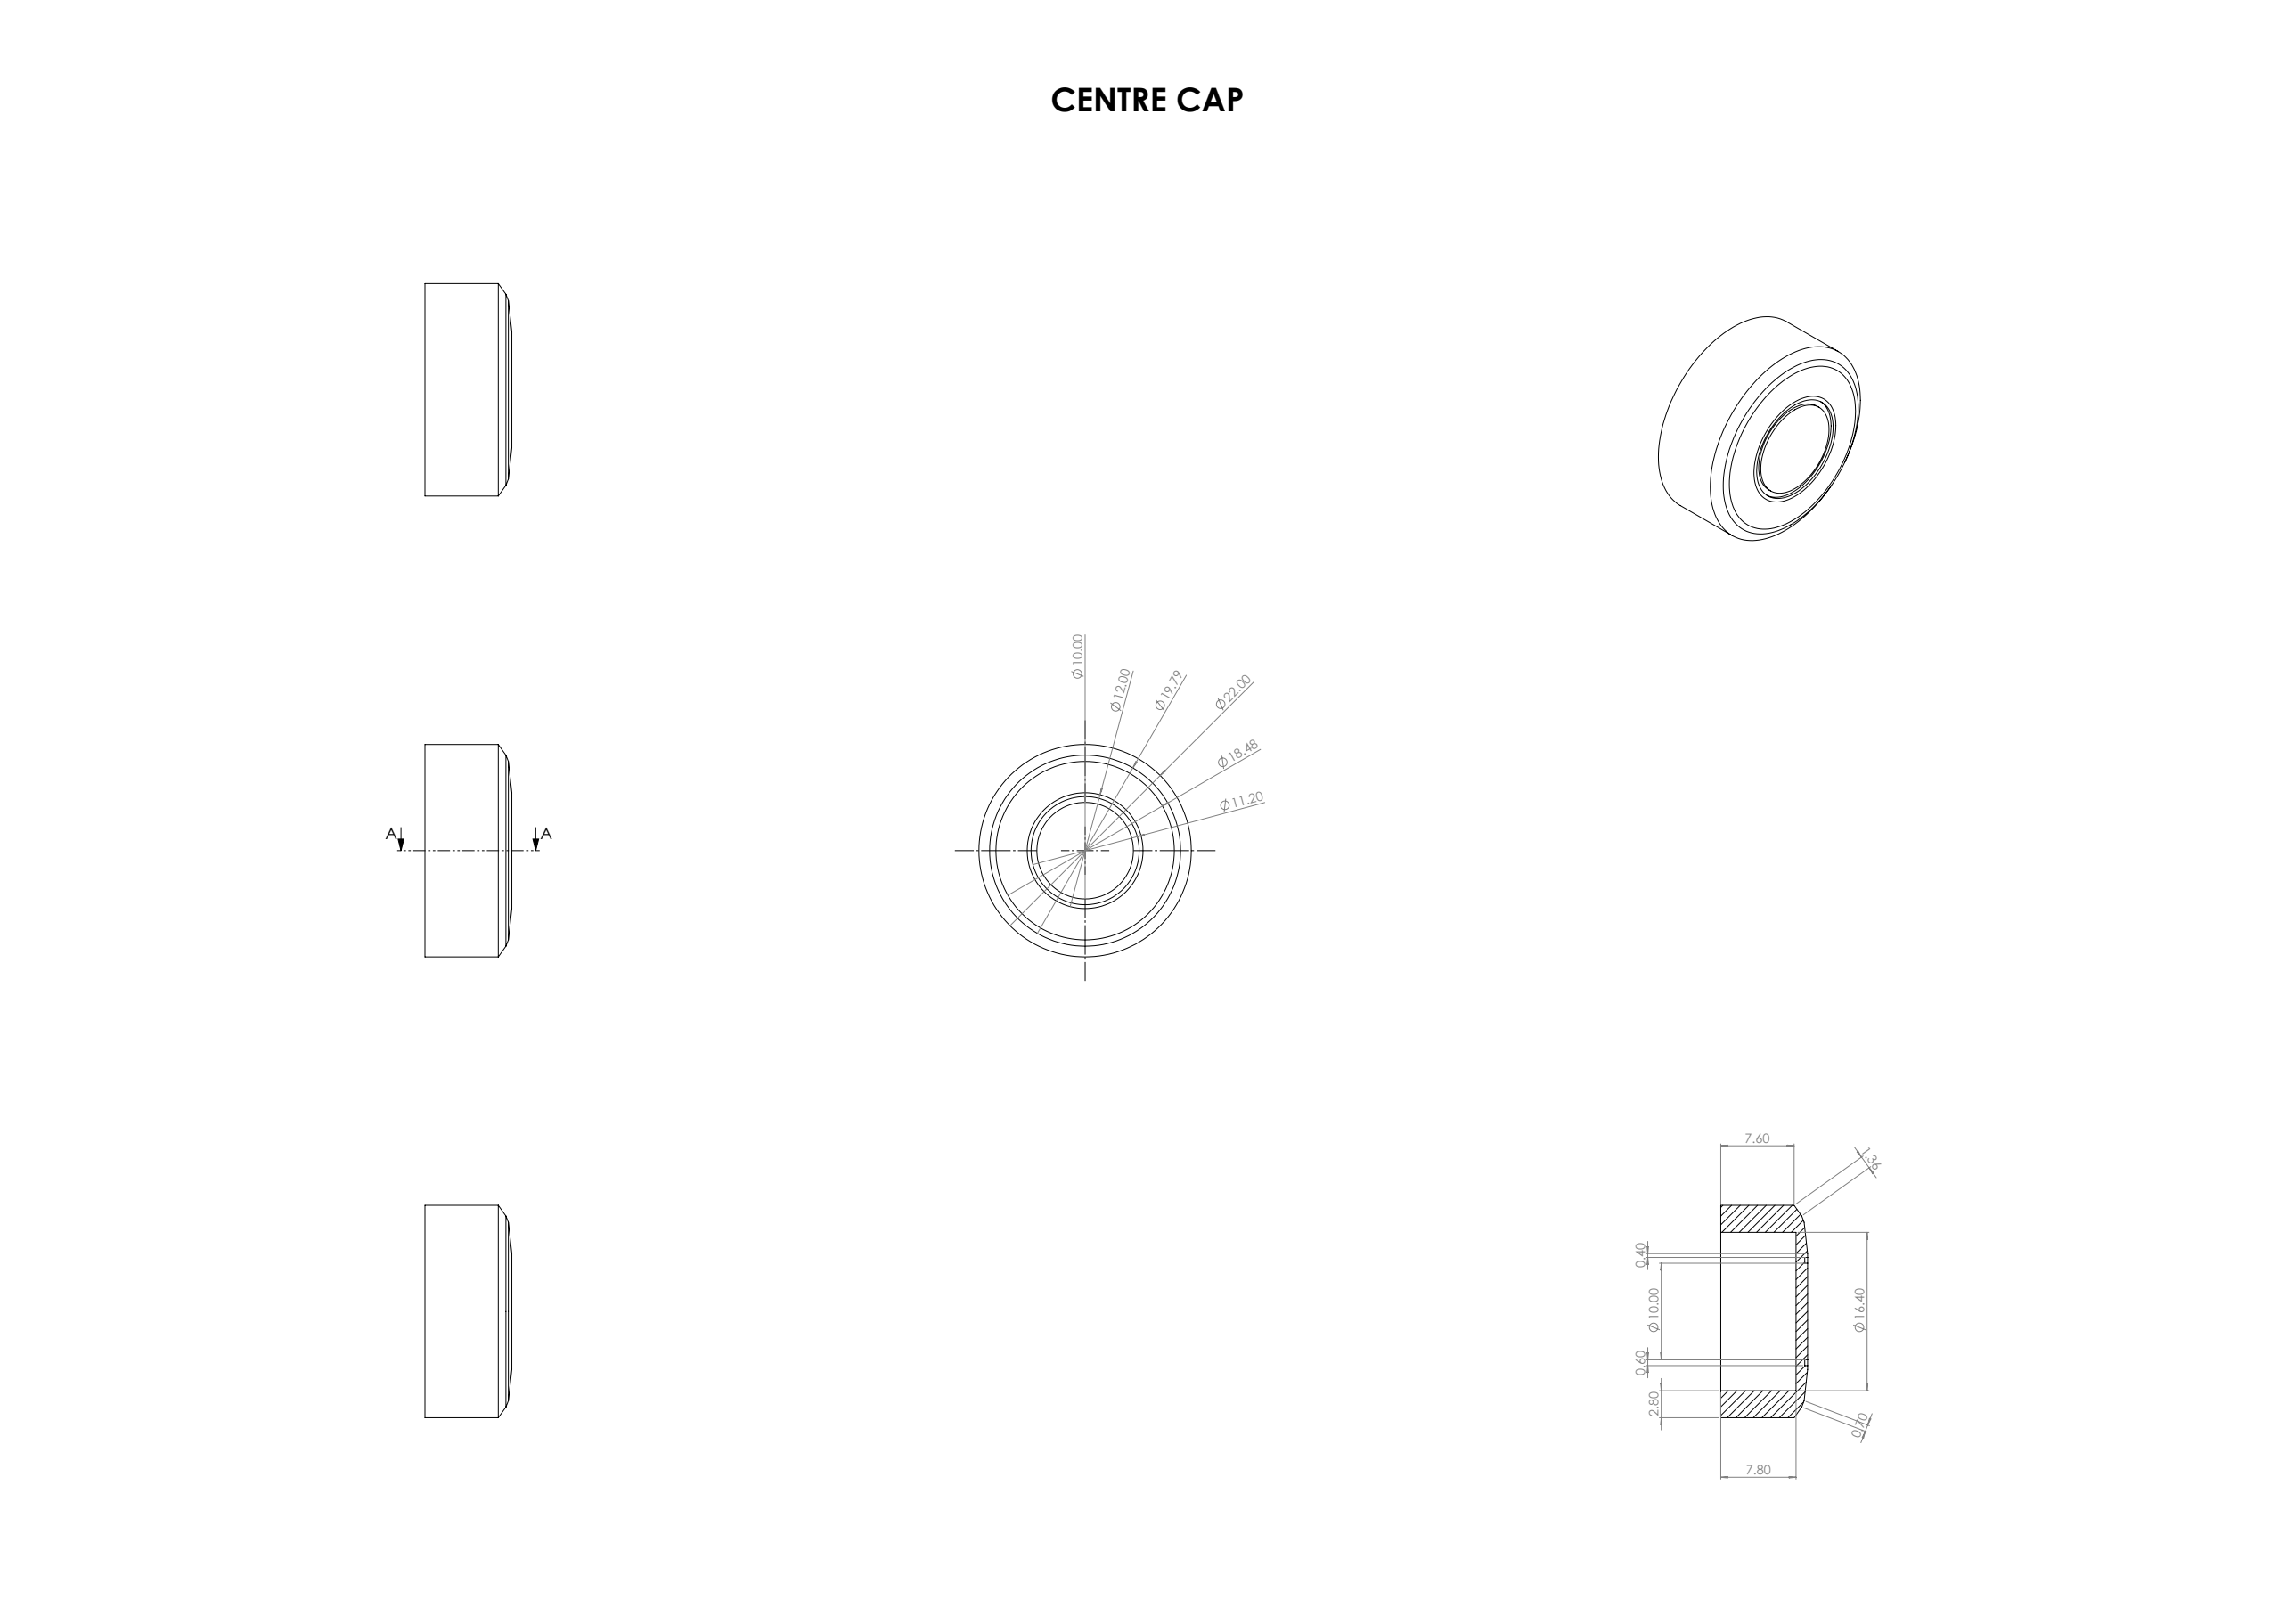
ISO-10303-21;
HEADER;
/* Generated by software containing ST-Developer
 * from STEP Tools, Inc. (www.steptools.com) 
 */

FILE_DESCRIPTION(
/* description */ (''),
/* implementation_level */ '2;1');

FILE_NAME(
/* name */ '05_Centre_Cap.step',
/* time_stamp */ '2026-10-21T02:03:06-07:00',
/* author */ (''),
/* organization */ (''),
/* preprocessor_version */ 'ST-DEVELOPER v20.2',
/* originating_system */ 'Autodesk Translation Framework v15.15.0.0',
/* authorisation */ '');

FILE_SCHEMA (('AUTOMOTIVE_DESIGN { 1 0 10303 214 3 1 1 }'));
ENDSEC;

DATA;
#10=MECHANICAL_DESIGN_GEOMETRIC_PRESENTATION_REPRESENTATION('',(#119),#38528);
#95=SHAPE_REPRESENTATION_RELATIONSHIP('SRR','None',#38580,#107);
#107=ADVANCED_BREP_SHAPE_REPRESENTATION('',(#131),#38520);
#119=STYLED_ITEM('',(#38692),#131);
#131=MANIFOLD_SOLID_BREP('Body1',#17076);
#377=CYLINDRICAL_SURFACE('',#18686,5.6);
#378=CYLINDRICAL_SURFACE('',#18688,5.);
#379=CYLINDRICAL_SURFACE('',#18691,8.2);
#380=CYLINDRICAL_SURFACE('',#18696,11.);
#1031=CONICAL_SURFACE('',#18674,9.56757295257596,1.20534297321654);
#1032=CONICAL_SURFACE('',#18679,10.3,0.950546840812076);
#1033=CONICAL_SURFACE('',#18681,7.8,1.460139105621);
#1466=FACE_BOUND('',#4065,.T.);
#1467=FACE_BOUND('',#4071,.T.);
#1468=FACE_BOUND('',#4074,.T.);
#2160=CIRCLE('',#18675,9.2422018555175);
#2161=CIRCLE('',#18676,9.2422018555175);
#2162=CIRCLE('',#18677,9.89294404963443);
#2163=CIRCLE('',#18678,9.89294404963443);
#2164=CIRCLE('',#18680,11.);
#2165=CIRCLE('',#18682,6.);
#2166=CIRCLE('',#18684,5.6);
#2167=CIRCLE('',#18685,5.);
#2168=CIRCLE('',#18687,5.6);
#2169=CIRCLE('',#18689,5.);
#2170=CIRCLE('',#18692,8.2);
#2171=CIRCLE('',#18693,8.2);
#2172=CIRCLE('',#18695,11.);
#3044=FACE_OUTER_BOUND('',#4061,.T.);
#3045=FACE_OUTER_BOUND('',#4062,.T.);
#3046=FACE_OUTER_BOUND('',#4063,.T.);
#3047=FACE_OUTER_BOUND('',#4064,.T.);
#3048=FACE_OUTER_BOUND('',#4066,.T.);
#3049=FACE_OUTER_BOUND('',#4067,.T.);
#3050=FACE_OUTER_BOUND('',#4068,.T.);
#3051=FACE_OUTER_BOUND('',#4069,.T.);
#3052=FACE_OUTER_BOUND('',#4070,.T.);
#3053=FACE_OUTER_BOUND('',#4072,.T.);
#3054=FACE_OUTER_BOUND('',#4073,.T.);
#3055=FACE_OUTER_BOUND('',#4075,.T.);
#4061=EDGE_LOOP('',(#14479,#14480,#14481,#14482,#14483,#14484));
#4062=EDGE_LOOP('',(#14485,#14486,#14487,#14488,#14489));
#4063=EDGE_LOOP('',(#14490,#14491,#14492,#14493,#14494));
#4064=EDGE_LOOP('',(#14495));
#4065=EDGE_LOOP('',(#14496));
#4066=EDGE_LOOP('',(#14497,#14498,#14499,#14500));
#4067=EDGE_LOOP('',(#14501,#14502,#14503,#14504));
#4068=EDGE_LOOP('',(#14505));
#4069=EDGE_LOOP('',(#14506,#14507,#14508,#14509));
#4070=EDGE_LOOP('',(#14510));
#4071=EDGE_LOOP('',(#14511));
#4072=EDGE_LOOP('',(#14512,#14513,#14514,#14515));
#4073=EDGE_LOOP('',(#14516));
#4074=EDGE_LOOP('',(#14517));
#4075=EDGE_LOOP('',(#14518));
#5019=LINE('',#33126,#5994);
#5020=LINE('',#33132,#5995);
#5021=LINE('',#33137,#5996);
#5022=LINE('',#33145,#5997);
#5023=LINE('',#33149,#5998);
#5024=LINE('',#33156,#5999);
#5025=LINE('',#33162,#6000);
#5994=VECTOR('',#22673,9.56757295257596);
#5995=VECTOR('',#22680,10.3);
#5996=VECTOR('',#22687,7.8);
#5997=VECTOR('',#22696,5.6);
#5998=VECTOR('',#22701,5.);
#5999=VECTOR('',#22710,8.2);
#6000=VECTOR('',#22719,11.);
#7511=VERTEX_POINT('',#33121);
#7512=VERTEX_POINT('',#33122);
#7513=VERTEX_POINT('',#33125);
#7514=VERTEX_POINT('',#33127);
#7515=VERTEX_POINT('',#33131);
#7516=VERTEX_POINT('',#33135);
#7517=VERTEX_POINT('',#33139);
#7518=VERTEX_POINT('',#33141);
#7519=VERTEX_POINT('',#33144);
#7520=VERTEX_POINT('',#33148);
#7521=VERTEX_POINT('',#33153);
#7522=VERTEX_POINT('',#33155);
#7523=VERTEX_POINT('',#33159);
#9891=EDGE_CURVE('',#7511,#7512,#2160,.T.);
#9892=EDGE_CURVE('',#7512,#7511,#2161,.T.);
#9893=EDGE_CURVE('',#7511,#7513,#5019,.T.);
#9894=EDGE_CURVE('',#7513,#7514,#2162,.T.);
#9895=EDGE_CURVE('',#7514,#7513,#2163,.T.);
#9896=EDGE_CURVE('',#7514,#7515,#5020,.T.);
#9897=EDGE_CURVE('',#7515,#7515,#2164,.T.);
#9898=EDGE_CURVE('',#7516,#7516,#2165,.T.);
#9899=EDGE_CURVE('',#7516,#7512,#5021,.T.);
#9900=EDGE_CURVE('',#7517,#7517,#2166,.T.);
#9901=EDGE_CURVE('',#7518,#7518,#2167,.T.);
#9902=EDGE_CURVE('',#7517,#7519,#5022,.T.);
#9903=EDGE_CURVE('',#7519,#7519,#2168,.T.);
#9904=EDGE_CURVE('',#7518,#7520,#5023,.T.);
#9905=EDGE_CURVE('',#7520,#7520,#2169,.T.);
#9906=EDGE_CURVE('',#7521,#7521,#2170,.T.);
#9907=EDGE_CURVE('',#7521,#7522,#5024,.T.);
#9908=EDGE_CURVE('',#7522,#7522,#2171,.T.);
#9909=EDGE_CURVE('',#7523,#7523,#2172,.T.);
#9910=EDGE_CURVE('',#7515,#7523,#5025,.T.);
#14479=ORIENTED_EDGE('',*,*,#9891,.T.);
#14480=ORIENTED_EDGE('',*,*,#9892,.T.);
#14481=ORIENTED_EDGE('',*,*,#9893,.T.);
#14482=ORIENTED_EDGE('',*,*,#9894,.T.);
#14483=ORIENTED_EDGE('',*,*,#9895,.T.);
#14484=ORIENTED_EDGE('',*,*,#9893,.F.);
#14485=ORIENTED_EDGE('',*,*,#9894,.F.);
#14486=ORIENTED_EDGE('',*,*,#9895,.F.);
#14487=ORIENTED_EDGE('',*,*,#9896,.T.);
#14488=ORIENTED_EDGE('',*,*,#9897,.T.);
#14489=ORIENTED_EDGE('',*,*,#9896,.F.);
#14490=ORIENTED_EDGE('',*,*,#9898,.F.);
#14491=ORIENTED_EDGE('',*,*,#9899,.T.);
#14492=ORIENTED_EDGE('',*,*,#9891,.F.);
#14493=ORIENTED_EDGE('',*,*,#9892,.F.);
#14494=ORIENTED_EDGE('',*,*,#9899,.F.);
#14495=ORIENTED_EDGE('',*,*,#9900,.T.);
#14496=ORIENTED_EDGE('',*,*,#9901,.F.);
#14497=ORIENTED_EDGE('',*,*,#9900,.F.);
#14498=ORIENTED_EDGE('',*,*,#9902,.T.);
#14499=ORIENTED_EDGE('',*,*,#9903,.F.);
#14500=ORIENTED_EDGE('',*,*,#9902,.F.);
#14501=ORIENTED_EDGE('',*,*,#9901,.T.);
#14502=ORIENTED_EDGE('',*,*,#9904,.T.);
#14503=ORIENTED_EDGE('',*,*,#9905,.F.);
#14504=ORIENTED_EDGE('',*,*,#9904,.F.);
#14505=ORIENTED_EDGE('',*,*,#9905,.T.);
#14506=ORIENTED_EDGE('',*,*,#9906,.T.);
#14507=ORIENTED_EDGE('',*,*,#9907,.T.);
#14508=ORIENTED_EDGE('',*,*,#9908,.F.);
#14509=ORIENTED_EDGE('',*,*,#9907,.F.);
#14510=ORIENTED_EDGE('',*,*,#9909,.F.);
#14511=ORIENTED_EDGE('',*,*,#9908,.T.);
#14512=ORIENTED_EDGE('',*,*,#9897,.F.);
#14513=ORIENTED_EDGE('',*,*,#9910,.T.);
#14514=ORIENTED_EDGE('',*,*,#9909,.T.);
#14515=ORIENTED_EDGE('',*,*,#9910,.F.);
#14516=ORIENTED_EDGE('',*,*,#9898,.T.);
#14517=ORIENTED_EDGE('',*,*,#9903,.T.);
#14518=ORIENTED_EDGE('',*,*,#9906,.F.);
#15953=PLANE('',#18683);
#15954=PLANE('',#18690);
#15955=PLANE('',#18694);
#15956=PLANE('',#18697);
#15957=PLANE('',#18698);
#16853=ADVANCED_FACE('',(#3044),#1031,.T.);
#16854=ADVANCED_FACE('',(#3045),#1032,.T.);
#16855=ADVANCED_FACE('',(#3046),#1033,.T.);
#16856=ADVANCED_FACE('',(#3047,#1466),#15953,.F.);
#16857=ADVANCED_FACE('',(#3048),#377,.F.);
#16858=ADVANCED_FACE('',(#3049),#378,.T.);
#16859=ADVANCED_FACE('',(#3050),#15954,.T.);
#16860=ADVANCED_FACE('',(#3051),#379,.F.);
#16861=ADVANCED_FACE('',(#3052,#1467),#15955,.T.);
#16862=ADVANCED_FACE('',(#3053),#380,.T.);
#16863=ADVANCED_FACE('',(#3054,#1468),#15956,.T.);
#16864=ADVANCED_FACE('',(#3055),#15957,.T.);
#17076=CLOSED_SHELL('',(#16853,#16854,#16855,#16856,#16857,#16858,#16859,
#16860,#16861,#16862,#16863,#16864));
#18673=AXIS2_PLACEMENT_3D('',#33119,#22665,#22666);
#18674=AXIS2_PLACEMENT_3D('',#33120,#22667,#22668);
#18675=AXIS2_PLACEMENT_3D('',#33123,#22669,#22670);
#18676=AXIS2_PLACEMENT_3D('',#33124,#22671,#22672);
#18677=AXIS2_PLACEMENT_3D('',#33128,#22674,#22675);
#18678=AXIS2_PLACEMENT_3D('',#33129,#22676,#22677);
#18679=AXIS2_PLACEMENT_3D('',#33130,#22678,#22679);
#18680=AXIS2_PLACEMENT_3D('',#33133,#22681,#22682);
#18681=AXIS2_PLACEMENT_3D('',#33134,#22683,#22684);
#18682=AXIS2_PLACEMENT_3D('',#33136,#22685,#22686);
#18683=AXIS2_PLACEMENT_3D('',#33138,#22688,#22689);
#18684=AXIS2_PLACEMENT_3D('',#33140,#22690,#22691);
#18685=AXIS2_PLACEMENT_3D('',#33142,#22692,#22693);
#18686=AXIS2_PLACEMENT_3D('',#33143,#22694,#22695);
#18687=AXIS2_PLACEMENT_3D('',#33146,#22697,#22698);
#18688=AXIS2_PLACEMENT_3D('',#33147,#22699,#22700);
#18689=AXIS2_PLACEMENT_3D('',#33150,#22702,#22703);
#18690=AXIS2_PLACEMENT_3D('',#33151,#22704,#22705);
#18691=AXIS2_PLACEMENT_3D('',#33152,#22706,#22707);
#18692=AXIS2_PLACEMENT_3D('',#33154,#22708,#22709);
#18693=AXIS2_PLACEMENT_3D('',#33157,#22711,#22712);
#18694=AXIS2_PLACEMENT_3D('',#33158,#22713,#22714);
#18695=AXIS2_PLACEMENT_3D('',#33160,#22715,#22716);
#18696=AXIS2_PLACEMENT_3D('',#33161,#22717,#22718);
#18697=AXIS2_PLACEMENT_3D('',#33163,#22720,#22721);
#18698=AXIS2_PLACEMENT_3D('',#33164,#22722,#22723);
#22665=DIRECTION('axis',(0.,0.,1.));
#22666=DIRECTION('refdir',(1.,0.,0.));
#22667=DIRECTION('center_axis',(-1.,0.,-1.6002526653361E-16));
#22668=DIRECTION('ref_axis',(0.,-1.,-6.12323399573677E-17));
#22669=DIRECTION('center_axis',(-1.,0.,0.));
#22670=DIRECTION('ref_axis',(0.,-1.,-6.12323399573677E-17));
#22671=DIRECTION('center_axis',(-1.,0.,0.));
#22672=DIRECTION('ref_axis',(0.,-1.,-6.12323399573677E-17));
#22673=DIRECTION('',(-0.35737274613036,0.933961840935295,1.14377337902718E-16));
#22674=DIRECTION('center_axis',(1.,0.,0.));
#22675=DIRECTION('ref_axis',(0.,-1.,-6.12323399573676E-17));
#22676=DIRECTION('center_axis',(1.,0.,0.));
#22677=DIRECTION('ref_axis',(0.,-1.,-6.12323399573676E-17));
#22678=DIRECTION('center_axis',(-1.,0.,0.));
#22679=DIRECTION('ref_axis',(0.,1.,0.));
#22680=DIRECTION('',(-0.581238193719096,-0.813733471206735,-9.96536090872393E-17));
#22681=DIRECTION('center_axis',(1.,0.,0.));
#22682=DIRECTION('ref_axis',(0.,0.,-1.));
#22683=DIRECTION('center_axis',(-1.,0.,0.));
#22684=DIRECTION('ref_axis',(0.,1.,0.));
#22685=DIRECTION('center_axis',(1.,0.,0.));
#22686=DIRECTION('ref_axis',(0.,0.,-1.));
#22687=DIRECTION('',(-0.110431526074847,-0.993883734673619,-1.21715653439266E-16));
#22688=DIRECTION('center_axis',(-1.,0.,0.));
#22689=DIRECTION('ref_axis',(0.,0.,1.));
#22690=DIRECTION('center_axis',(1.,0.,0.));
#22691=DIRECTION('ref_axis',(0.,0.,-1.));
#22692=DIRECTION('center_axis',(1.,0.,0.));
#22693=DIRECTION('ref_axis',(0.,0.,-1.));
#22694=DIRECTION('center_axis',(1.,0.,0.));
#22695=DIRECTION('ref_axis',(0.,1.,0.));
#22696=DIRECTION('',(1.,0.,0.));
#22697=DIRECTION('center_axis',(-1.,0.,0.));
#22698=DIRECTION('ref_axis',(0.,1.,0.));
#22699=DIRECTION('center_axis',(1.,0.,0.));
#22700=DIRECTION('ref_axis',(0.,1.,0.));
#22701=DIRECTION('',(1.,0.,0.));
#22702=DIRECTION('center_axis',(1.,0.,0.));
#22703=DIRECTION('ref_axis',(0.,1.,0.));
#22704=DIRECTION('center_axis',(1.,0.,0.));
#22705=DIRECTION('ref_axis',(0.,0.,-1.));
#22706=DIRECTION('center_axis',(1.,0.,0.));
#22707=DIRECTION('ref_axis',(0.,1.,0.));
#22708=DIRECTION('center_axis',(1.,0.,0.));
#22709=DIRECTION('ref_axis',(0.,0.,-1.));
#22710=DIRECTION('',(-1.,0.,0.));
#22711=DIRECTION('center_axis',(1.,0.,0.));
#22712=DIRECTION('ref_axis',(0.,0.,-1.));
#22713=DIRECTION('center_axis',(-1.,0.,0.));
#22714=DIRECTION('ref_axis',(0.,0.,1.));
#22715=DIRECTION('center_axis',(1.,0.,0.));
#22716=DIRECTION('ref_axis',(0.,0.,-1.));
#22717=DIRECTION('center_axis',(1.,0.,0.));
#22718=DIRECTION('ref_axis',(0.,1.,0.));
#22719=DIRECTION('',(-1.,0.,0.));
#22720=DIRECTION('center_axis',(1.,0.,0.));
#22721=DIRECTION('ref_axis',(0.,0.,-1.));
#22722=DIRECTION('center_axis',(-1.,0.,0.));
#22723=DIRECTION('ref_axis',(0.,0.,1.));
#33119=CARTESIAN_POINT('',(0.,0.,0.));
#33120=CARTESIAN_POINT('Origin',(8.51525479982404,0.,-5.85844879599047E-16));
#33121=CARTESIAN_POINT('',(8.63975534938695,9.2422018555175,-1.13184329194332E-15));
#33122=CARTESIAN_POINT('',(8.63975534938694,-9.2422018555175,-1.13184329194332E-15));
#33123=CARTESIAN_POINT('Origin',(8.63975534938695,0.,-5.65921645971662E-16));
#33124=CARTESIAN_POINT('Origin',(8.63975534938695,0.,-5.65921645971662E-16));
#33125=CARTESIAN_POINT('',(8.39075425026112,9.89294404963443,1.21153622645287E-15));
#33126=CARTESIAN_POINT('',(8.51525479982404,9.56757295257596,1.17168975919809E-15));
#33127=CARTESIAN_POINT('',(8.39075425026113,-9.89294404963442,-1.21153622645287E-15));
#33128=CARTESIAN_POINT('Origin',(8.39075425026112,0.,-6.05768113226433E-16));
#33129=CARTESIAN_POINT('Origin',(8.39075425026112,0.,-6.05768113226433E-16));
#33130=CARTESIAN_POINT('Origin',(8.1,0.,0.));
#33131=CARTESIAN_POINT('',(7.6,-11.,-1.34711147906209E-15));
#33132=CARTESIAN_POINT('',(8.1,-10.3,-1.26138620312177E-15));
#33133=CARTESIAN_POINT('Origin',(7.6,0.,0.));
#33134=CARTESIAN_POINT('Origin',(8.8,0.,0.));
#33135=CARTESIAN_POINT('',(9.,-6.,-7.34788079488412E-16));
#33136=CARTESIAN_POINT('Origin',(9.,0.,0.));
#33137=CARTESIAN_POINT('',(8.8,-7.8,-9.55224503334935E-16));
#33138=CARTESIAN_POINT('Origin',(8.7,5.6,0.));
#33139=CARTESIAN_POINT('',(8.7,-5.6,-6.85802207522518E-16));
#33140=CARTESIAN_POINT('Origin',(8.7,0.,0.));
#33141=CARTESIAN_POINT('',(8.7,-5.,-6.12323399573677E-16));
#33142=CARTESIAN_POINT('Origin',(8.7,0.,0.));
#33143=CARTESIAN_POINT('Origin',(8.855,0.,0.));
#33144=CARTESIAN_POINT('',(9.,-5.6,6.85802207522518E-16));
#33145=CARTESIAN_POINT('',(8.855,-5.6,-6.85802207522518E-16));
#33146=CARTESIAN_POINT('Origin',(9.,0.,0.));
#33147=CARTESIAN_POINT('Origin',(8.855,0.,0.));
#33148=CARTESIAN_POINT('',(9.,-5.,-6.12323399573677E-16));
#33149=CARTESIAN_POINT('',(8.855,-5.,-6.12323399573677E-16));
#33150=CARTESIAN_POINT('Origin',(9.,0.,0.));
#33151=CARTESIAN_POINT('Origin',(9.,0.,0.));
#33152=CARTESIAN_POINT('Origin',(3.9,0.,0.));
#33153=CARTESIAN_POINT('',(7.8,-8.2,-1.00421037530083E-15));
#33154=CARTESIAN_POINT('Origin',(7.8,0.,0.));
#33155=CARTESIAN_POINT('',(0.,-8.2,-1.00421037530083E-15));
#33156=CARTESIAN_POINT('',(3.9,-8.2,-1.00421037530083E-15));
#33157=CARTESIAN_POINT('Origin',(0.,0.,0.));
#33158=CARTESIAN_POINT('Origin',(0.,11.,0.));
#33159=CARTESIAN_POINT('',(5.55111512312578E-16,-11.,-1.34711147906209E-15));
#33160=CARTESIAN_POINT('Origin',(0.,0.,0.));
#33161=CARTESIAN_POINT('Origin',(3.8,0.,0.));
#33162=CARTESIAN_POINT('',(3.8,-11.,-1.34711147906209E-15));
#33163=CARTESIAN_POINT('Origin',(9.,0.,0.));
#33164=CARTESIAN_POINT('Origin',(7.8,8.2,0.));
#38506=UNCERTAINTY_MEASURE_WITH_UNIT(LENGTH_MEASURE(0.01),#38529,
'DISTANCE_ACCURACY_VALUE',
'Maximum model space distance between geometric entities at asserted c
onnectivities');
#38514=UNCERTAINTY_MEASURE_WITH_UNIT(LENGTH_MEASURE(0.01),#38529,
'DISTANCE_ACCURACY_VALUE',
'Maximum model space distance between geometric entities at asserted c
onnectivities');
#38520=(
GEOMETRIC_REPRESENTATION_CONTEXT(3)
GLOBAL_UNCERTAINTY_ASSIGNED_CONTEXT((#38506))
GLOBAL_UNIT_ASSIGNED_CONTEXT((#38529,#38531,#38532))
REPRESENTATION_CONTEXT('','3D')
);
#38528=(
GEOMETRIC_REPRESENTATION_CONTEXT(3)
GLOBAL_UNCERTAINTY_ASSIGNED_CONTEXT((#38514))
GLOBAL_UNIT_ASSIGNED_CONTEXT((#38529,#38531,#38532))
REPRESENTATION_CONTEXT('','3D')
);
#38529=(
LENGTH_UNIT()
NAMED_UNIT(*)
SI_UNIT(.MILLI.,.METRE.)
);
#38531=(
NAMED_UNIT(*)
PLANE_ANGLE_UNIT()
SI_UNIT($,.RADIAN.)
);
#38532=(
NAMED_UNIT(*)
SI_UNIT($,.STERADIAN.)
SOLID_ANGLE_UNIT()
);
#38538=SHAPE_DEFINITION_REPRESENTATION(#38551,#38580);
#38551=PRODUCT_DEFINITION_SHAPE('',$,#38594);
#38580=SHAPE_REPRESENTATION('',(#18673),#38520);
#38588=PRODUCT_DEFINITION_CONTEXT('part definition',#38629,'design');
#38594=PRODUCT_DEFINITION('2026-10-20-13-39-08-542','05_Centre_Cap',#38607,
#38588);
#38607=PRODUCT_DEFINITION_FORMATION('',$,#38636);
#38629=APPLICATION_CONTEXT(
'Core Data for Automotive Mechanical Design Process');
#38630=PRODUCT_CONTEXT('part definition',#38629,'mechanical');
#38636=PRODUCT('2026-10-20-13-39-08-542','05_Centre_Cap',$,(#38630));
#38686=COLOUR_RGB('Light Blue',0.38,0.62,0.78);
#38687=FILL_AREA_STYLE_COLOUR('',#38686);
#38688=FILL_AREA_STYLE('',(#38687));
#38689=SURFACE_STYLE_FILL_AREA(#38688);
#38690=SURFACE_SIDE_STYLE('',(#38689));
#38691=SURFACE_STYLE_USAGE(.BOTH.,#38690);
#38692=PRESENTATION_STYLE_ASSIGNMENT((#38691));
ENDSEC;
END-ISO-10303-21;
